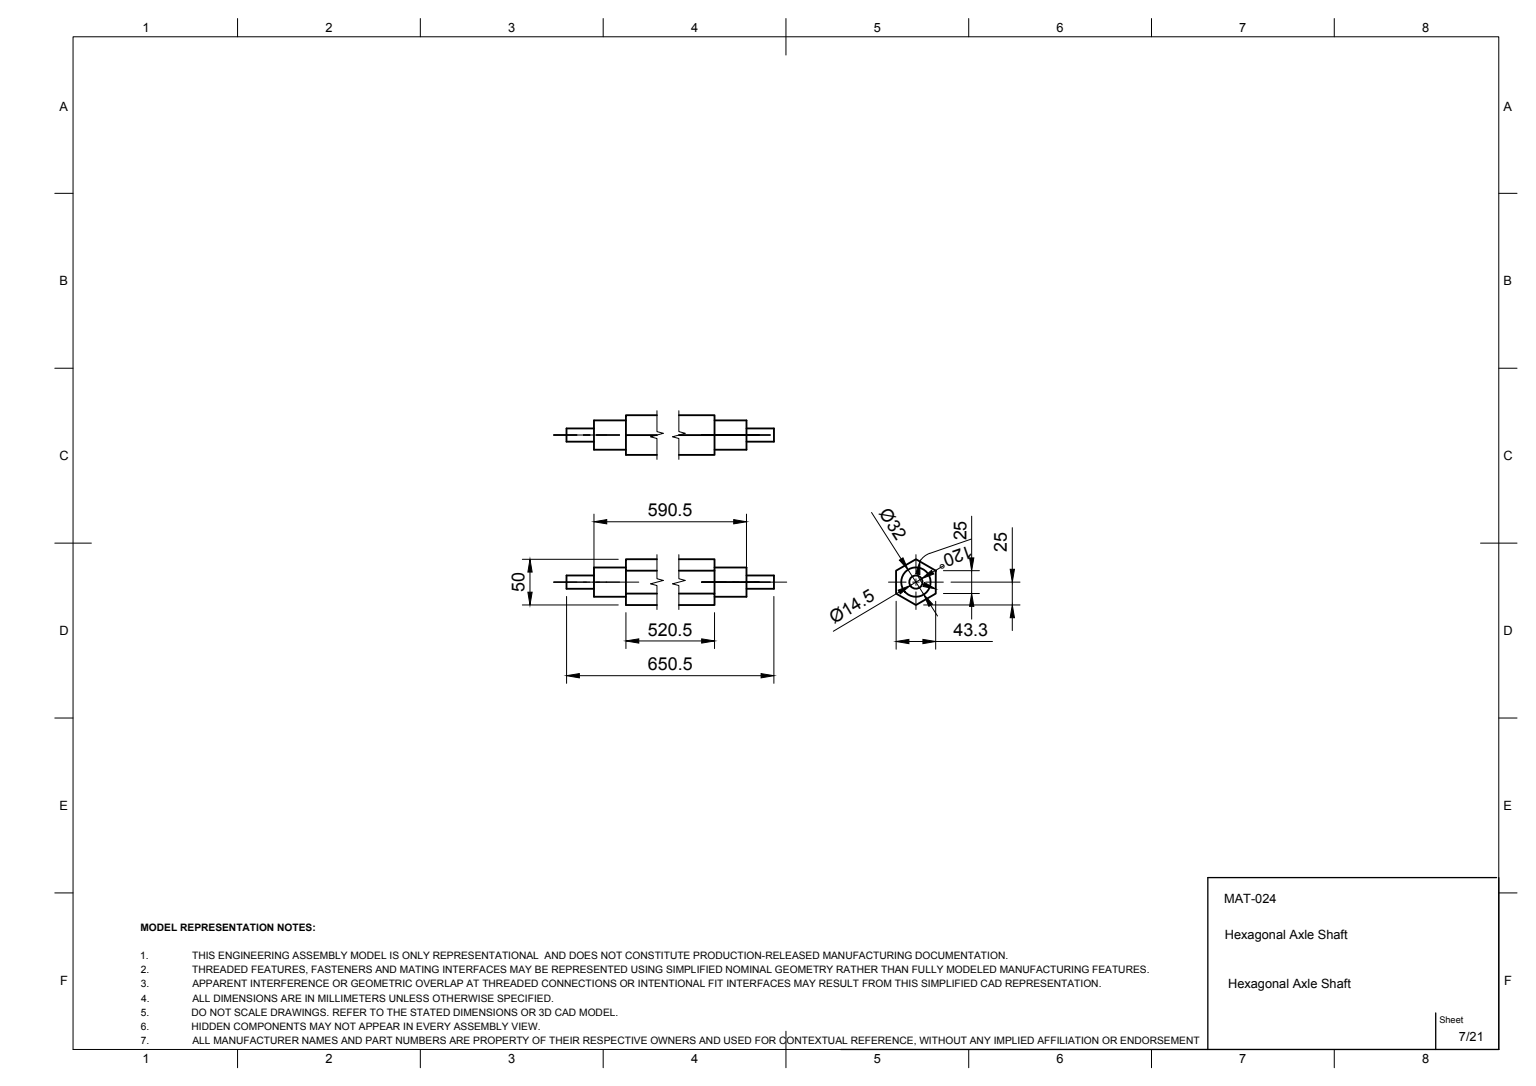
ISO-10303-21;
HEADER;
/* Generated by software containing ST-Developer
 * from STEP Tools, Inc. (www.steptools.com) 
 */

FILE_DESCRIPTION(
/* description */ ('STEP AP214'),
/* implementation_level */ '2;1');

FILE_NAME(
/* name */ 'Hexagonal Axle Shaft.step',
/* time_stamp */ '2026-11-14T06:34:07-08:00',
/* author */ (''),
/* organization */ (''),
/* preprocessor_version */ 'ST-DEVELOPER v20.2',
/* originating_system */ 'Autodesk Translation Framework v15.17.0.0',
/* authorisation */ '');

FILE_SCHEMA (('AUTOMOTIVE_DESIGN { 1 0 10303 214 3 1 1 }'));
ENDSEC;

DATA;
#10=MECHANICAL_DESIGN_GEOMETRIC_PRESENTATION_REPRESENTATION('',(#7313),#310623);
#7231=SHAPE_REPRESENTATION_RELATIONSHIP('SRR','None',#310904,#7248);
#7248=ADVANCED_BREP_SHAPE_REPRESENTATION('',(#7381),#310613);
#7313=STYLED_ITEM('',(#311007),#7381);
#7381=MANIFOLD_SOLID_BREP('Body1',#93763);
#7648=FACE_BOUND('',#20009,.T.);
#7649=FACE_BOUND('',#20011,.T.);
#7650=FACE_BOUND('',#20013,.T.);
#7651=FACE_BOUND('',#20016,.T.);
#8557=PLANE('',#104236);
#8558=PLANE('',#104237);
#8559=PLANE('',#104238);
#8560=PLANE('',#104239);
#8561=PLANE('',#104240);
#8562=PLANE('',#104241);
#8563=PLANE('',#104242);
#8564=PLANE('',#104243);
#8565=PLANE('',#104244);
#8566=PLANE('',#104245);
#8567=PLANE('',#104246);
#8568=PLANE('',#104247);
#14002=FACE_OUTER_BOUND('',#19998,.T.);
#14003=FACE_OUTER_BOUND('',#19999,.T.);
#14004=FACE_OUTER_BOUND('',#20000,.T.);
#14005=FACE_OUTER_BOUND('',#20001,.T.);
#14006=FACE_OUTER_BOUND('',#20002,.T.);
#14007=FACE_OUTER_BOUND('',#20003,.T.);
#14008=FACE_OUTER_BOUND('',#20004,.T.);
#14009=FACE_OUTER_BOUND('',#20005,.T.);
#14010=FACE_OUTER_BOUND('',#20006,.T.);
#14011=FACE_OUTER_BOUND('',#20007,.T.);
#14012=FACE_OUTER_BOUND('',#20008,.T.);
#14013=FACE_OUTER_BOUND('',#20010,.T.);
#14014=FACE_OUTER_BOUND('',#20012,.T.);
#14015=FACE_OUTER_BOUND('',#20014,.T.);
#14016=FACE_OUTER_BOUND('',#20015,.T.);
#14017=FACE_OUTER_BOUND('',#20017,.T.);
#19998=EDGE_LOOP('',(#83655,#83656,#83657,#83658));
#19999=EDGE_LOOP('',(#83659,#83660,#83661,#83662));
#20000=EDGE_LOOP('',(#83663,#83664,#83665,#83666));
#20001=EDGE_LOOP('',(#83667,#83668,#83669,#83670));
#20002=EDGE_LOOP('',(#83671,#83672,#83673,#83674));
#20003=EDGE_LOOP('',(#83675,#83676,#83677,#83678));
#20004=EDGE_LOOP('',(#83679,#83680,#83681,#83682));
#20005=EDGE_LOOP('',(#83683,#83684,#83685,#83686));
#20006=EDGE_LOOP('',(#83687,#83688,#83689,#83690));
#20007=EDGE_LOOP('',(#83691,#83692,#83693,#83694));
#20008=EDGE_LOOP('',(#83695,#83696,#83697,#83698,#83699,#83700));
#20009=EDGE_LOOP('',(#83701));
#20010=EDGE_LOOP('',(#83702,#83703,#83704,#83705,#83706,#83707));
#20011=EDGE_LOOP('',(#83708));
#20012=EDGE_LOOP('',(#83709));
#20013=EDGE_LOOP('',(#83710));
#20014=EDGE_LOOP('',(#83711));
#20015=EDGE_LOOP('',(#83712));
#20016=EDGE_LOOP('',(#83713));
#20017=EDGE_LOOP('',(#83714));
#24440=LINE('',#275497,#28787);
#24441=LINE('',#275503,#28788);
#24442=LINE('',#275509,#28789);
#24443=LINE('',#275515,#28790);
#24444=LINE('',#275520,#28791);
#24445=LINE('',#275522,#28792);
#24446=LINE('',#275524,#28793);
#24447=LINE('',#275525,#28794);
#24448=LINE('',#275528,#28795);
#24449=LINE('',#275530,#28796);
#24450=LINE('',#275531,#28797);
#24451=LINE('',#275534,#28798);
#24452=LINE('',#275536,#28799);
#24453=LINE('',#275537,#28800);
#24454=LINE('',#275540,#28801);
#24455=LINE('',#275542,#28802);
#24456=LINE('',#275543,#28803);
#24457=LINE('',#275546,#28804);
#24458=LINE('',#275548,#28805);
#24459=LINE('',#275549,#28806);
#24460=LINE('',#275551,#28807);
#24461=LINE('',#275552,#28808);
#28787=VECTOR('',#129349,7.25);
#28788=VECTOR('',#129356,16.);
#28789=VECTOR('',#129363,7.25);
#28790=VECTOR('',#129370,16.);
#28791=VECTOR('',#129375,1000.);
#28792=VECTOR('',#129376,1000.);
#28793=VECTOR('',#129377,1000.);
#28794=VECTOR('',#129378,1000.);
#28795=VECTOR('',#129381,1000.);
#28796=VECTOR('',#129382,1000.);
#28797=VECTOR('',#129383,1000.);
#28798=VECTOR('',#129386,1000.);
#28799=VECTOR('',#129387,1000.);
#28800=VECTOR('',#129388,1000.);
#28801=VECTOR('',#129391,1000.);
#28802=VECTOR('',#129392,1000.);
#28803=VECTOR('',#129393,1000.);
#28804=VECTOR('',#129396,1000.);
#28805=VECTOR('',#129397,1000.);
#28806=VECTOR('',#129398,1000.);
#28807=VECTOR('',#129401,1000.);
#28808=VECTOR('',#129402,1000.);
#34938=CIRCLE('',#104225,7.25);
#34939=CIRCLE('',#104226,7.25);
#34940=CIRCLE('',#104228,16.);
#34941=CIRCLE('',#104229,16.);
#34942=CIRCLE('',#104231,7.25);
#34943=CIRCLE('',#104232,7.25);
#34944=CIRCLE('',#104234,16.);
#34945=CIRCLE('',#104235,16.);
#42929=VERTEX_POINT('',#275494);
#42930=VERTEX_POINT('',#275496);
#42931=VERTEX_POINT('',#275500);
#42932=VERTEX_POINT('',#275502);
#42933=VERTEX_POINT('',#275506);
#42934=VERTEX_POINT('',#275508);
#42935=VERTEX_POINT('',#275512);
#42936=VERTEX_POINT('',#275514);
#42937=VERTEX_POINT('',#275518);
#42938=VERTEX_POINT('',#275519);
#42939=VERTEX_POINT('',#275521);
#42940=VERTEX_POINT('',#275523);
#42941=VERTEX_POINT('',#275527);
#42942=VERTEX_POINT('',#275529);
#42943=VERTEX_POINT('',#275533);
#42944=VERTEX_POINT('',#275535);
#42945=VERTEX_POINT('',#275539);
#42946=VERTEX_POINT('',#275541);
#42947=VERTEX_POINT('',#275545);
#42948=VERTEX_POINT('',#275547);
#56607=EDGE_CURVE('',#42929,#42929,#34938,.T.);
#56608=EDGE_CURVE('',#42929,#42930,#24440,.T.);
#56609=EDGE_CURVE('',#42930,#42930,#34939,.T.);
#56610=EDGE_CURVE('',#42931,#42931,#34940,.T.);
#56611=EDGE_CURVE('',#42931,#42932,#24441,.T.);
#56612=EDGE_CURVE('',#42932,#42932,#34941,.T.);
#56613=EDGE_CURVE('',#42933,#42933,#34942,.T.);
#56614=EDGE_CURVE('',#42933,#42934,#24442,.T.);
#56615=EDGE_CURVE('',#42934,#42934,#34943,.T.);
#56616=EDGE_CURVE('',#42935,#42935,#34944,.T.);
#56617=EDGE_CURVE('',#42935,#42936,#24443,.T.);
#56618=EDGE_CURVE('',#42936,#42936,#34945,.T.);
#56619=EDGE_CURVE('',#42937,#42938,#24444,.T.);
#56620=EDGE_CURVE('',#42939,#42938,#24445,.T.);
#56621=EDGE_CURVE('',#42940,#42939,#24446,.T.);
#56622=EDGE_CURVE('',#42940,#42937,#24447,.T.);
#56623=EDGE_CURVE('',#42938,#42941,#24448,.T.);
#56624=EDGE_CURVE('',#42942,#42941,#24449,.T.);
#56625=EDGE_CURVE('',#42939,#42942,#24450,.T.);
#56626=EDGE_CURVE('',#42941,#42943,#24451,.T.);
#56627=EDGE_CURVE('',#42944,#42943,#24452,.T.);
#56628=EDGE_CURVE('',#42942,#42944,#24453,.T.);
#56629=EDGE_CURVE('',#42943,#42945,#24454,.T.);
#56630=EDGE_CURVE('',#42946,#42945,#24455,.T.);
#56631=EDGE_CURVE('',#42944,#42946,#24456,.T.);
#56632=EDGE_CURVE('',#42945,#42947,#24457,.T.);
#56633=EDGE_CURVE('',#42948,#42947,#24458,.T.);
#56634=EDGE_CURVE('',#42946,#42948,#24459,.T.);
#56635=EDGE_CURVE('',#42947,#42937,#24460,.T.);
#56636=EDGE_CURVE('',#42948,#42940,#24461,.T.);
#83655=ORIENTED_EDGE('',*,*,#56607,.F.);
#83656=ORIENTED_EDGE('',*,*,#56608,.T.);
#83657=ORIENTED_EDGE('',*,*,#56609,.T.);
#83658=ORIENTED_EDGE('',*,*,#56608,.F.);
#83659=ORIENTED_EDGE('',*,*,#56610,.F.);
#83660=ORIENTED_EDGE('',*,*,#56611,.T.);
#83661=ORIENTED_EDGE('',*,*,#56612,.T.);
#83662=ORIENTED_EDGE('',*,*,#56611,.F.);
#83663=ORIENTED_EDGE('',*,*,#56613,.T.);
#83664=ORIENTED_EDGE('',*,*,#56614,.T.);
#83665=ORIENTED_EDGE('',*,*,#56615,.F.);
#83666=ORIENTED_EDGE('',*,*,#56614,.F.);
#83667=ORIENTED_EDGE('',*,*,#56616,.T.);
#83668=ORIENTED_EDGE('',*,*,#56617,.T.);
#83669=ORIENTED_EDGE('',*,*,#56618,.F.);
#83670=ORIENTED_EDGE('',*,*,#56617,.F.);
#83671=ORIENTED_EDGE('',*,*,#56619,.T.);
#83672=ORIENTED_EDGE('',*,*,#56620,.F.);
#83673=ORIENTED_EDGE('',*,*,#56621,.F.);
#83674=ORIENTED_EDGE('',*,*,#56622,.T.);
#83675=ORIENTED_EDGE('',*,*,#56623,.T.);
#83676=ORIENTED_EDGE('',*,*,#56624,.F.);
#83677=ORIENTED_EDGE('',*,*,#56625,.F.);
#83678=ORIENTED_EDGE('',*,*,#56620,.T.);
#83679=ORIENTED_EDGE('',*,*,#56626,.T.);
#83680=ORIENTED_EDGE('',*,*,#56627,.F.);
#83681=ORIENTED_EDGE('',*,*,#56628,.F.);
#83682=ORIENTED_EDGE('',*,*,#56624,.T.);
#83683=ORIENTED_EDGE('',*,*,#56629,.T.);
#83684=ORIENTED_EDGE('',*,*,#56630,.F.);
#83685=ORIENTED_EDGE('',*,*,#56631,.F.);
#83686=ORIENTED_EDGE('',*,*,#56627,.T.);
#83687=ORIENTED_EDGE('',*,*,#56632,.T.);
#83688=ORIENTED_EDGE('',*,*,#56633,.F.);
#83689=ORIENTED_EDGE('',*,*,#56634,.F.);
#83690=ORIENTED_EDGE('',*,*,#56630,.T.);
#83691=ORIENTED_EDGE('',*,*,#56635,.T.);
#83692=ORIENTED_EDGE('',*,*,#56622,.F.);
#83693=ORIENTED_EDGE('',*,*,#56636,.F.);
#83694=ORIENTED_EDGE('',*,*,#56633,.T.);
#83695=ORIENTED_EDGE('',*,*,#56621,.T.);
#83696=ORIENTED_EDGE('',*,*,#56625,.T.);
#83697=ORIENTED_EDGE('',*,*,#56628,.T.);
#83698=ORIENTED_EDGE('',*,*,#56631,.T.);
#83699=ORIENTED_EDGE('',*,*,#56634,.T.);
#83700=ORIENTED_EDGE('',*,*,#56636,.T.);
#83701=ORIENTED_EDGE('',*,*,#56616,.F.);
#83702=ORIENTED_EDGE('',*,*,#56619,.F.);
#83703=ORIENTED_EDGE('',*,*,#56635,.F.);
#83704=ORIENTED_EDGE('',*,*,#56632,.F.);
#83705=ORIENTED_EDGE('',*,*,#56629,.F.);
#83706=ORIENTED_EDGE('',*,*,#56626,.F.);
#83707=ORIENTED_EDGE('',*,*,#56623,.F.);
#83708=ORIENTED_EDGE('',*,*,#56610,.T.);
#83709=ORIENTED_EDGE('',*,*,#56618,.T.);
#83710=ORIENTED_EDGE('',*,*,#56613,.F.);
#83711=ORIENTED_EDGE('',*,*,#56615,.T.);
#83712=ORIENTED_EDGE('',*,*,#56612,.F.);
#83713=ORIENTED_EDGE('',*,*,#56607,.T.);
#83714=ORIENTED_EDGE('',*,*,#56609,.F.);
#87783=CYLINDRICAL_SURFACE('',#104224,7.25);
#87784=CYLINDRICAL_SURFACE('',#104227,16.);
#87785=CYLINDRICAL_SURFACE('',#104230,7.25);
#87786=CYLINDRICAL_SURFACE('',#104233,16.);
#93281=ADVANCED_FACE('',(#14002),#87783,.T.);
#93282=ADVANCED_FACE('',(#14003),#87784,.T.);
#93283=ADVANCED_FACE('',(#14004),#87785,.T.);
#93284=ADVANCED_FACE('',(#14005),#87786,.T.);
#93285=ADVANCED_FACE('',(#14006),#8557,.F.);
#93286=ADVANCED_FACE('',(#14007),#8558,.F.);
#93287=ADVANCED_FACE('',(#14008),#8559,.F.);
#93288=ADVANCED_FACE('',(#14009),#8560,.F.);
#93289=ADVANCED_FACE('',(#14010),#8561,.F.);
#93290=ADVANCED_FACE('',(#14011),#8562,.F.);
#93291=ADVANCED_FACE('',(#14012,#7648),#8563,.T.);
#93292=ADVANCED_FACE('',(#14013,#7649),#8564,.F.);
#93293=ADVANCED_FACE('',(#14014,#7650),#8565,.T.);
#93294=ADVANCED_FACE('',(#14015),#8566,.T.);
#93295=ADVANCED_FACE('',(#14016,#7651),#8567,.T.);
#93296=ADVANCED_FACE('',(#14017),#8568,.T.);
#93763=CLOSED_SHELL('',(#93281,#93282,#93283,#93284,#93285,#93286,#93287,
#93288,#93289,#93290,#93291,#93292,#93293,#93294,#93295,#93296));
#104223=AXIS2_PLACEMENT_3D('',#275492,#129343,#129344);
#104224=AXIS2_PLACEMENT_3D('',#275493,#129345,#129346);
#104225=AXIS2_PLACEMENT_3D('',#275495,#129347,#129348);
#104226=AXIS2_PLACEMENT_3D('',#275498,#129350,#129351);
#104227=AXIS2_PLACEMENT_3D('',#275499,#129352,#129353);
#104228=AXIS2_PLACEMENT_3D('',#275501,#129354,#129355);
#104229=AXIS2_PLACEMENT_3D('',#275504,#129357,#129358);
#104230=AXIS2_PLACEMENT_3D('',#275505,#129359,#129360);
#104231=AXIS2_PLACEMENT_3D('',#275507,#129361,#129362);
#104232=AXIS2_PLACEMENT_3D('',#275510,#129364,#129365);
#104233=AXIS2_PLACEMENT_3D('',#275511,#129366,#129367);
#104234=AXIS2_PLACEMENT_3D('',#275513,#129368,#129369);
#104235=AXIS2_PLACEMENT_3D('',#275516,#129371,#129372);
#104236=AXIS2_PLACEMENT_3D('',#275517,#129373,#129374);
#104237=AXIS2_PLACEMENT_3D('',#275526,#129379,#129380);
#104238=AXIS2_PLACEMENT_3D('',#275532,#129384,#129385);
#104239=AXIS2_PLACEMENT_3D('',#275538,#129389,#129390);
#104240=AXIS2_PLACEMENT_3D('',#275544,#129394,#129395);
#104241=AXIS2_PLACEMENT_3D('',#275550,#129399,#129400);
#104242=AXIS2_PLACEMENT_3D('',#275553,#129403,#129404);
#104243=AXIS2_PLACEMENT_3D('',#275554,#129405,#129406);
#104244=AXIS2_PLACEMENT_3D('',#275555,#129407,#129408);
#104245=AXIS2_PLACEMENT_3D('',#275556,#129409,#129410);
#104246=AXIS2_PLACEMENT_3D('',#275557,#129411,#129412);
#104247=AXIS2_PLACEMENT_3D('',#275558,#129413,#129414);
#129343=DIRECTION('axis',(0.,0.,1.));
#129344=DIRECTION('refdir',(1.,0.,0.));
#129345=DIRECTION('center_axis',(0.,0.,1.));
#129346=DIRECTION('ref_axis',(1.,0.,0.));
#129347=DIRECTION('center_axis',(0.,0.,1.));
#129348=DIRECTION('ref_axis',(1.,0.,0.));
#129349=DIRECTION('',(0.,0.,-1.));
#129350=DIRECTION('center_axis',(0.,0.,1.));
#129351=DIRECTION('ref_axis',(1.,0.,0.));
#129352=DIRECTION('center_axis',(0.,0.,1.));
#129353=DIRECTION('ref_axis',(1.,0.,0.));
#129354=DIRECTION('center_axis',(0.,0.,1.));
#129355=DIRECTION('ref_axis',(1.,0.,0.));
#129356=DIRECTION('',(0.,0.,-1.));
#129357=DIRECTION('center_axis',(0.,0.,1.));
#129358=DIRECTION('ref_axis',(1.,0.,0.));
#129359=DIRECTION('center_axis',(0.,0.,-1.));
#129360=DIRECTION('ref_axis',(-1.,0.,0.));
#129361=DIRECTION('center_axis',(0.,0.,1.));
#129362=DIRECTION('ref_axis',(1.,0.,0.));
#129363=DIRECTION('',(0.,0.,1.));
#129364=DIRECTION('center_axis',(0.,0.,1.));
#129365=DIRECTION('ref_axis',(1.,0.,0.));
#129366=DIRECTION('center_axis',(0.,0.,-1.));
#129367=DIRECTION('ref_axis',(-1.,0.,0.));
#129368=DIRECTION('center_axis',(0.,0.,1.));
#129369=DIRECTION('ref_axis',(1.,0.,0.));
#129370=DIRECTION('',(0.,0.,1.));
#129371=DIRECTION('center_axis',(0.,0.,1.));
#129372=DIRECTION('ref_axis',(1.,0.,0.));
#129373=DIRECTION('center_axis',(-0.5,-0.866025403784439,0.));
#129374=DIRECTION('ref_axis',(0.866025403784439,-0.5,0.));
#129375=DIRECTION('',(-0.866025403784439,0.5,0.));
#129376=DIRECTION('',(0.,0.,-1.));
#129377=DIRECTION('',(-0.866025403784439,0.5,0.));
#129378=DIRECTION('',(0.,0.,-1.));
#129379=DIRECTION('center_axis',(0.5,-0.866025403784439,0.));
#129380=DIRECTION('ref_axis',(0.866025403784439,0.5,0.));
#129381=DIRECTION('',(-0.866025403784439,-0.5,0.));
#129382=DIRECTION('',(0.,0.,-1.));
#129383=DIRECTION('',(-0.866025403784439,-0.5,0.));
#129384=DIRECTION('center_axis',(1.,1.38777878078145E-16,0.));
#129385=DIRECTION('ref_axis',(-1.38777878078145E-16,1.,0.));
#129386=DIRECTION('',(1.38777878078145E-16,-1.,0.));
#129387=DIRECTION('',(0.,0.,-1.));
#129388=DIRECTION('',(1.38777878078145E-16,-1.,0.));
#129389=DIRECTION('center_axis',(0.5,0.866025403784439,0.));
#129390=DIRECTION('ref_axis',(-0.866025403784439,0.5,0.));
#129391=DIRECTION('',(0.866025403784438,-0.5,0.));
#129392=DIRECTION('',(0.,0.,-1.));
#129393=DIRECTION('',(0.866025403784438,-0.5,0.));
#129394=DIRECTION('center_axis',(-0.5,0.866025403784439,0.));
#129395=DIRECTION('ref_axis',(-0.866025403784439,-0.5,0.));
#129396=DIRECTION('',(0.866025403784439,0.5,0.));
#129397=DIRECTION('',(0.,0.,-1.));
#129398=DIRECTION('',(0.866025403784439,0.5,0.));
#129399=DIRECTION('center_axis',(-1.,-1.38777878078144E-16,0.));
#129400=DIRECTION('ref_axis',(1.38777878078145E-16,-1.,0.));
#129401=DIRECTION('',(-1.38777878078144E-16,1.,0.));
#129402=DIRECTION('',(-1.38777878078144E-16,1.,0.));
#129403=DIRECTION('center_axis',(0.,0.,1.));
#129404=DIRECTION('ref_axis',(1.,0.,0.));
#129405=DIRECTION('center_axis',(0.,0.,1.));
#129406=DIRECTION('ref_axis',(1.,0.,0.));
#129407=DIRECTION('center_axis',(0.,0.,1.));
#129408=DIRECTION('ref_axis',(1.,0.,0.));
#129409=DIRECTION('center_axis',(0.,0.,1.));
#129410=DIRECTION('ref_axis',(1.,0.,0.));
#129411=DIRECTION('center_axis',(0.,0.,-1.));
#129412=DIRECTION('ref_axis',(1.,0.,0.));
#129413=DIRECTION('center_axis',(0.,0.,-1.));
#129414=DIRECTION('ref_axis',(1.,0.,0.));
#275492=CARTESIAN_POINT('',(0.,0.,0.));
#275493=CARTESIAN_POINT('Origin',(0.,0.,-325.25));
#275494=CARTESIAN_POINT('',(-7.25,-8.87868929381831E-16,-295.25));
#275495=CARTESIAN_POINT('Origin',(0.,0.,-295.25));
#275496=CARTESIAN_POINT('',(-7.25,-8.87868929381831E-16,-325.25));
#275497=CARTESIAN_POINT('',(-7.25,-8.87868929381831E-16,-325.25));
#275498=CARTESIAN_POINT('Origin',(0.,0.,-325.25));
#275499=CARTESIAN_POINT('Origin',(0.,0.,-295.25));
#275500=CARTESIAN_POINT('',(-16.,-1.95943487863577E-15,-260.25));
#275501=CARTESIAN_POINT('Origin',(0.,0.,-260.25));
#275502=CARTESIAN_POINT('',(-16.,-1.95943487863577E-15,-295.25));
#275503=CARTESIAN_POINT('',(-16.,-1.95943487863577E-15,-295.25));
#275504=CARTESIAN_POINT('Origin',(0.,0.,-295.25));
#275505=CARTESIAN_POINT('Origin',(0.,0.,325.25));
#275506=CARTESIAN_POINT('',(7.25,-8.87868929381831E-16,295.25));
#275507=CARTESIAN_POINT('Origin',(0.,0.,295.25));
#275508=CARTESIAN_POINT('',(7.25,-8.87868929381831E-16,325.25));
#275509=CARTESIAN_POINT('',(7.25,-8.87868929381831E-16,325.25));
#275510=CARTESIAN_POINT('Origin',(0.,0.,325.25));
#275511=CARTESIAN_POINT('Origin',(0.,0.,295.25));
#275512=CARTESIAN_POINT('',(16.,-1.95943487863577E-15,260.25));
#275513=CARTESIAN_POINT('Origin',(0.,0.,260.25));
#275514=CARTESIAN_POINT('',(16.,-1.95943487863577E-15,295.25));
#275515=CARTESIAN_POINT('',(16.,-1.95943487863577E-15,295.25));
#275516=CARTESIAN_POINT('Origin',(0.,0.,295.25));
#275517=CARTESIAN_POINT('Origin',(21.650635094611,12.5,260.25));
#275518=CARTESIAN_POINT('',(21.650635094611,12.5,-260.25));
#275519=CARTESIAN_POINT('',(3.0046291974743E-15,25.,-260.25));
#275520=CARTESIAN_POINT('',(21.650635094611,12.5,-260.25));
#275521=CARTESIAN_POINT('',(3.0046291974743E-15,25.,260.25));
#275522=CARTESIAN_POINT('',(3.0046291974743E-15,25.,260.25));
#275523=CARTESIAN_POINT('',(21.650635094611,12.5,260.25));
#275524=CARTESIAN_POINT('',(21.650635094611,12.5,260.25));
#275525=CARTESIAN_POINT('',(21.650635094611,12.5,260.25));
#275526=CARTESIAN_POINT('Origin',(3.0046291974743E-15,25.,260.25));
#275527=CARTESIAN_POINT('',(-21.650635094611,12.5,-260.25));
#275528=CARTESIAN_POINT('',(3.0046291974743E-15,25.,-260.25));
#275529=CARTESIAN_POINT('',(-21.650635094611,12.5,260.25));
#275530=CARTESIAN_POINT('',(-21.650635094611,12.5,260.25));
#275531=CARTESIAN_POINT('',(3.0046291974743E-15,25.,260.25));
#275532=CARTESIAN_POINT('Origin',(-21.650635094611,12.5,260.25));
#275533=CARTESIAN_POINT('',(-21.650635094611,-12.5,-260.25));
#275534=CARTESIAN_POINT('',(-21.650635094611,12.5,-260.25));
#275535=CARTESIAN_POINT('',(-21.650635094611,-12.5,260.25));
#275536=CARTESIAN_POINT('',(-21.650635094611,-12.5,260.25));
#275537=CARTESIAN_POINT('',(-21.650635094611,12.5,260.25));
#275538=CARTESIAN_POINT('Origin',(-21.650635094611,-12.5,260.25));
#275539=CARTESIAN_POINT('',(3.87537447643023E-16,-25.,-260.25));
#275540=CARTESIAN_POINT('',(-21.650635094611,-12.5,-260.25));
#275541=CARTESIAN_POINT('',(3.87537447643023E-16,-25.,260.25));
#275542=CARTESIAN_POINT('',(3.87537447643023E-16,-25.,260.25));
#275543=CARTESIAN_POINT('',(-21.650635094611,-12.5,260.25));
#275544=CARTESIAN_POINT('Origin',(3.87537447643023E-16,-25.,260.25));
#275545=CARTESIAN_POINT('',(21.650635094611,-12.5,-260.25));
#275546=CARTESIAN_POINT('',(3.87537447643023E-16,-25.,-260.25));
#275547=CARTESIAN_POINT('',(21.650635094611,-12.5,260.25));
#275548=CARTESIAN_POINT('',(21.650635094611,-12.5,260.25));
#275549=CARTESIAN_POINT('',(3.87537447643023E-16,-25.,260.25));
#275550=CARTESIAN_POINT('Origin',(21.650635094611,-12.5,260.25));
#275551=CARTESIAN_POINT('',(21.650635094611,-12.5,-260.25));
#275552=CARTESIAN_POINT('',(21.650635094611,-12.5,260.25));
#275553=CARTESIAN_POINT('Origin',(0.,0.,260.25));
#275554=CARTESIAN_POINT('Origin',(0.,0.,-260.25));
#275555=CARTESIAN_POINT('Origin',(0.,0.,295.25));
#275556=CARTESIAN_POINT('Origin',(0.,0.,325.25));
#275557=CARTESIAN_POINT('Origin',(0.,0.,-295.25));
#275558=CARTESIAN_POINT('Origin',(0.,0.,-325.25));
#310591=UNCERTAINTY_MEASURE_WITH_UNIT(LENGTH_MEASURE(0.01),#310624,
'DISTANCE_ACCURACY_VALUE',
'Maximum model space distance between geometric entities at asserted c
onnectivities');
#310601=UNCERTAINTY_MEASURE_WITH_UNIT(LENGTH_MEASURE(0.01),#310624,
'DISTANCE_ACCURACY_VALUE',
'Maximum model space distance between geometric entities at asserted c
onnectivities');
#310613=(
GEOMETRIC_REPRESENTATION_CONTEXT(3)
GLOBAL_UNCERTAINTY_ASSIGNED_CONTEXT((#310591))
GLOBAL_UNIT_ASSIGNED_CONTEXT((#310624,#310626,#310627))
REPRESENTATION_CONTEXT('','3D')
);
#310623=(
GEOMETRIC_REPRESENTATION_CONTEXT(3)
GLOBAL_UNCERTAINTY_ASSIGNED_CONTEXT((#310601))
GLOBAL_UNIT_ASSIGNED_CONTEXT((#310624,#310626,#310627))
REPRESENTATION_CONTEXT('','3D')
);
#310624=(
LENGTH_UNIT()
NAMED_UNIT(*)
SI_UNIT(.MILLI.,.METRE.)
);
#310626=(
NAMED_UNIT(*)
PLANE_ANGLE_UNIT()
SI_UNIT($,.RADIAN.)
);
#310627=(
NAMED_UNIT(*)
SI_UNIT($,.STERADIAN.)
SOLID_ANGLE_UNIT()
);
#310639=SHAPE_DEFINITION_REPRESENTATION(#310798,#310904);
#310798=PRODUCT_DEFINITION_SHAPE('',$,#310926);
#310904=SHAPE_REPRESENTATION('',(#104223),#310613);
#310914=PRODUCT_DEFINITION_CONTEXT('part definition',#310979,'design');
#310926=PRODUCT_DEFINITION('Hexagonal Axle Shaft',
'Hexagonal Axle Shaft',#310947,#310914);
#310947=PRODUCT_DEFINITION_FORMATION('',$,#310992);
#310979=APPLICATION_CONTEXT(
'Core Data for Automotive Mechanical Design Process');
#310980=PRODUCT_CONTEXT('part definition',#310979,'mechanical');
#310992=PRODUCT('Hexagonal Axle Shaft','Hexagonal Axle Shaft',$,(#310980));
#311007=PRESENTATION_STYLE_ASSIGNMENT((#311014));
#311014=SURFACE_STYLE_USAGE(.BOTH.,#311021);
#311021=SURFACE_SIDE_STYLE('',(#311028));
#311028=SURFACE_STYLE_FILL_AREA(#311035);
#311035=FILL_AREA_STYLE('Opaque(122,133,145)',(#311042));
#311042=FILL_AREA_STYLE_COLOUR('Opaque(122,133,145)',#311049);
#311049=COLOUR_RGB('Opaque(122,133,145)',0.47843137254902,0.52156862745098,
0.568627450980392);
ENDSEC;
END-ISO-10303-21;
